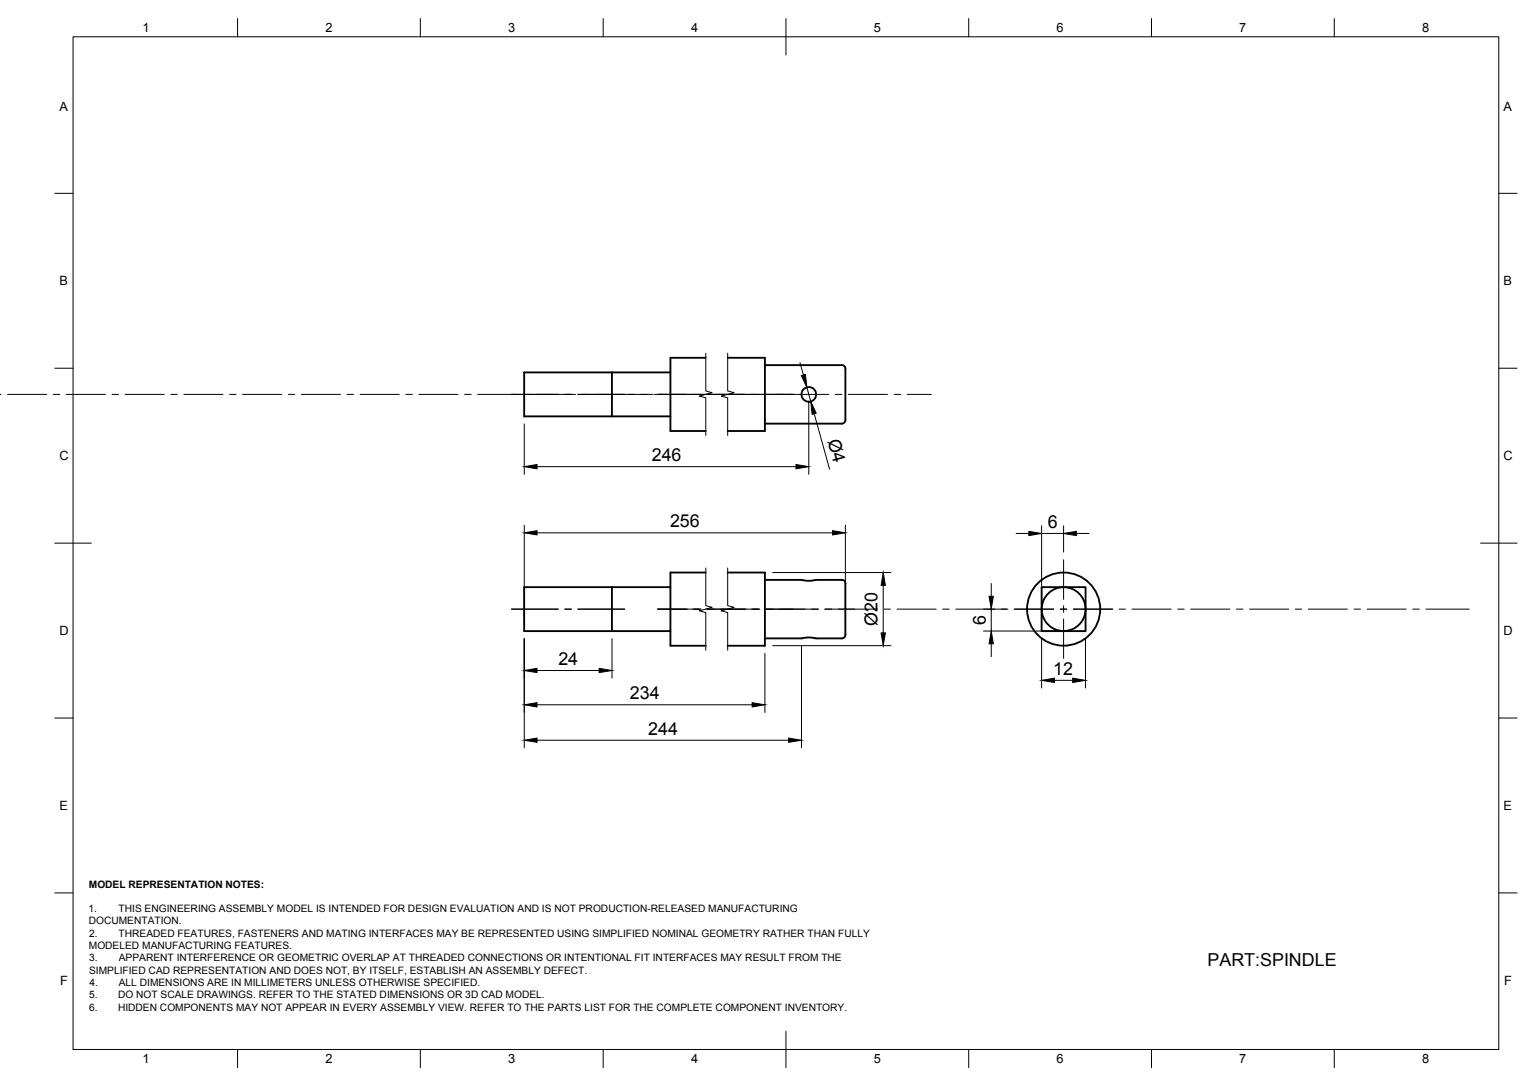
ISO-10303-21;
HEADER;
/* Generated by software containing ST-Developer
 * from STEP Tools, Inc. (www.steptools.com) 
 */

FILE_DESCRIPTION(
/* description */ (''),
/* implementation_level */ '2;1');

FILE_NAME(
/* name */ 'SPINDLE.step',
/* time_stamp */ '2026-10-04T02:10:06-07:00',
/* author */ (''),
/* organization */ (''),
/* preprocessor_version */ 'ST-DEVELOPER v20.2',
/* originating_system */ 'Autodesk Translation Framework v15.15.0.0',
/* authorisation */ '');

FILE_SCHEMA (('AUTOMOTIVE_DESIGN { 1 0 10303 214 3 1 1 }'));
ENDSEC;

DATA;
#10=MECHANICAL_DESIGN_GEOMETRIC_PRESENTATION_REPRESENTATION('',(#143),#9668);
#121=SHAPE_REPRESENTATION_RELATIONSHIP('SRR','None',#9714,#132);
#132=ADVANCED_BREP_SHAPE_REPRESENTATION('',(#154),#9659);
#143=STYLED_ITEM('',(#9775),#154);
#154=MANIFOLD_SOLID_BREP('Body1',#3883);
#233=FACE_BOUND('',#1154,.T.);
#234=FACE_BOUND('',#1157,.T.);
#235=FACE_BOUND('',#1159,.T.);
#236=FACE_BOUND('',#1160,.T.);
#299=PLANE('',#4195);
#300=PLANE('',#4197);
#301=PLANE('',#4199);
#302=PLANE('',#4201);
#303=PLANE('',#4203);
#304=PLANE('',#4207);
#305=PLANE('',#4214);
#306=PLANE('',#4215);
#307=PLANE('',#4216);
#308=PLANE('',#4217);
#309=PLANE('',#4218);
#310=PLANE('',#4222);
#446=LINE('',#6435,#637);
#447=LINE('',#6436,#638);
#448=LINE('',#6441,#639);
#449=LINE('',#6442,#640);
#450=LINE('',#6447,#641);
#451=LINE('',#6448,#642);
#452=LINE('',#6457,#643);
#453=LINE('',#6459,#644);
#454=LINE('',#6461,#645);
#455=LINE('',#6462,#646);
#456=LINE('',#6466,#647);
#457=LINE('',#6473,#648);
#458=LINE('',#6551,#649);
#459=LINE('',#6555,#650);
#460=LINE('',#6557,#651);
#461=LINE('',#6558,#652);
#462=LINE('',#6560,#653);
#463=LINE('',#6562,#654);
#464=LINE('',#6564,#655);
#465=LINE('',#6569,#656);
#637=VECTOR('',#4910,6.);
#638=VECTOR('',#4911,6.);
#639=VECTOR('',#4916,6.);
#640=VECTOR('',#4917,6.);
#641=VECTOR('',#4922,6.);
#642=VECTOR('',#4923,6.);
#643=VECTOR('',#4932,12.);
#644=VECTOR('',#4933,12.);
#645=VECTOR('',#4934,12.);
#646=VECTOR('',#4935,12.);
#647=VECTOR('',#4940,9.99999999999998);
#648=VECTOR('',#4949,8.);
#649=VECTOR('',#4952,2.);
#650=VECTOR('',#4959,16.);
#651=VECTOR('',#4960,6.);
#652=VECTOR('',#4961,16.);
#653=VECTOR('',#4964,16.);
#654=VECTOR('',#4967,16.);
#655=VECTOR('',#4970,6.);
#656=VECTOR('',#4977,6.);
#786=CYLINDRICAL_SURFACE('',#4205,9.99999999999998);
#787=CYLINDRICAL_SURFACE('',#4209,8.);
#788=CYLINDRICAL_SURFACE('',#4211,2.);
#789=CYLINDRICAL_SURFACE('',#4220,6.);
#888=FACE_OUTER_BOUND('',#1149,.T.);
#889=FACE_OUTER_BOUND('',#1150,.T.);
#890=FACE_OUTER_BOUND('',#1151,.T.);
#891=FACE_OUTER_BOUND('',#1152,.T.);
#892=FACE_OUTER_BOUND('',#1153,.T.);
#893=FACE_OUTER_BOUND('',#1155,.T.);
#894=FACE_OUTER_BOUND('',#1156,.T.);
#895=FACE_OUTER_BOUND('',#1158,.T.);
#896=FACE_OUTER_BOUND('',#1161,.T.);
#897=FACE_OUTER_BOUND('',#1162,.T.);
#898=FACE_OUTER_BOUND('',#1163,.T.);
#899=FACE_OUTER_BOUND('',#1164,.T.);
#900=FACE_OUTER_BOUND('',#1165,.T.);
#901=FACE_OUTER_BOUND('',#1166,.T.);
#902=FACE_OUTER_BOUND('',#1167,.T.);
#903=FACE_OUTER_BOUND('',#1168,.T.);
#904=FACE_OUTER_BOUND('',#1169,.T.);
#1149=EDGE_LOOP('',(#2933,#2934,#2935));
#1150=EDGE_LOOP('',(#2936,#2937,#2938));
#1151=EDGE_LOOP('',(#2939,#2940,#2941));
#1152=EDGE_LOOP('',(#2942));
#1153=EDGE_LOOP('',(#2943));
#1154=EDGE_LOOP('',(#2944,#2945,#2946,#2947));
#1155=EDGE_LOOP('',(#2948,#2949,#2950,#2951));
#1156=EDGE_LOOP('',(#2952));
#1157=EDGE_LOOP('',(#2953));
#1158=EDGE_LOOP('',(#2954,#2955,#2956,#2957));
#1159=EDGE_LOOP('',(#2958,#2959));
#1160=EDGE_LOOP('',(#2960,#2961));
#1161=EDGE_LOOP('',(#2962,#2963,#2964,#2965,#2966,#2967));
#1162=EDGE_LOOP('',(#2968,#2969,#2970,#2971));
#1163=EDGE_LOOP('',(#2972,#2973,#2974,#2975,#2976));
#1164=EDGE_LOOP('',(#2977,#2978,#2979,#2980,#2981));
#1165=EDGE_LOOP('',(#2982,#2983,#2984,#2985,#2986));
#1166=EDGE_LOOP('',(#2987,#2988,#2989,#2990,#2991));
#1167=EDGE_LOOP('',(#2992,#2993,#2994));
#1168=EDGE_LOOP('',(#2995,#2996,#2997,#2998,#2999,#3000,#3001));
#1169=EDGE_LOOP('',(#3002));
#1343=B_SPLINE_CURVE_WITH_KNOTS('',3,(#6476,#6477,#6478,#6479,#6480,#6481,
#6482,#6483,#6484,#6485,#6486,#6487,#6488,#6489,#6490,#6491,#6492,#6493),
 .UNSPECIFIED.,.F.,.F.,(4,2,2,2,2,2,2,2,4),(0.605474840211907,0.681164486618941,
0.756854133025976,0.832533196671918,0.90821226031786,0.983891323963802,
1.05957038760974,1.13526003401678,1.21094968042381),.UNSPECIFIED.);
#1344=B_SPLINE_CURVE_WITH_KNOTS('',3,(#6494,#6495,#6496,#6497,#6498,#6499,
#6500,#6501,#6502,#6503,#6504,#6505,#6506,#6507,#6508,#6509,#6510,#6511),
 .UNSPECIFIED.,.F.,.F.,(4,2,2,2,2,2,2,2,4),(1.21094968042381,1.28663932683085,
1.36232897323788,1.43800803688382,1.51368710052977,1.58936616417571,1.66504522782165,
1.74073487422869,1.81642452063572),.UNSPECIFIED.);
#1345=B_SPLINE_CURVE_WITH_KNOTS('',3,(#6514,#6515,#6516,#6517,#6518,#6519,
#6520,#6521,#6522,#6523,#6524,#6525,#6526,#6527,#6528,#6529,#6530,#6531),
 .UNSPECIFIED.,.F.,.F.,(4,2,2,2,2,2,2,2,4),(0.605474840211907,0.681164486618941,
0.756854133025976,0.832533196671918,0.90821226031786,0.983891323963802,
1.05957038760974,1.13526003401678,1.21094968042381),.UNSPECIFIED.);
#1346=B_SPLINE_CURVE_WITH_KNOTS('',3,(#6532,#6533,#6534,#6535,#6536,#6537,
#6538,#6539,#6540,#6541,#6542,#6543,#6544,#6545,#6546,#6547,#6548,#6549),
 .UNSPECIFIED.,.F.,.F.,(4,2,2,2,2,2,2,2,4),(1.21094968042381,1.28663932683085,
1.36232897323788,1.43800803688382,1.51368710052977,1.58936616417571,1.66504522782165,
1.74073487422869,1.81642452063572),.UNSPECIFIED.);
#1526=CIRCLE('',#4196,6.);
#1527=CIRCLE('',#4198,6.);
#1528=CIRCLE('',#4200,6.);
#1529=CIRCLE('',#4202,7.);
#1530=CIRCLE('',#4204,9.99999999999995);
#1531=CIRCLE('',#4206,10.);
#1532=CIRCLE('',#4208,7.99999999999999);
#1533=CIRCLE('',#4210,8.);
#1534=CIRCLE('',#4213,1.);
#1535=CIRCLE('',#4219,6.);
#1536=CIRCLE('',#4221,6.);
#1769=VERTEX_POINT('',#6431);
#1770=VERTEX_POINT('',#6432);
#1771=VERTEX_POINT('',#6434);
#1772=VERTEX_POINT('',#6438);
#1773=VERTEX_POINT('',#6440);
#1774=VERTEX_POINT('',#6444);
#1775=VERTEX_POINT('',#6446);
#1776=VERTEX_POINT('',#6450);
#1777=VERTEX_POINT('',#6453);
#1778=VERTEX_POINT('',#6455);
#1779=VERTEX_POINT('',#6456);
#1780=VERTEX_POINT('',#6458);
#1781=VERTEX_POINT('',#6460);
#1782=VERTEX_POINT('',#6464);
#1783=VERTEX_POINT('',#6468);
#1784=VERTEX_POINT('',#6471);
#1785=VERTEX_POINT('',#6474);
#1786=VERTEX_POINT('',#6475);
#1787=VERTEX_POINT('',#6512);
#1788=VERTEX_POINT('',#6513);
#1789=VERTEX_POINT('',#6556);
#1790=VERTEX_POINT('',#6568);
#2190=EDGE_CURVE('',#1769,#1770,#1526,.T.);
#2191=EDGE_CURVE('',#1769,#1771,#446,.T.);
#2192=EDGE_CURVE('',#1771,#1770,#447,.T.);
#2193=EDGE_CURVE('',#1770,#1772,#1527,.T.);
#2194=EDGE_CURVE('',#1770,#1773,#448,.T.);
#2195=EDGE_CURVE('',#1773,#1772,#449,.T.);
#2196=EDGE_CURVE('',#1772,#1774,#1528,.T.);
#2197=EDGE_CURVE('',#1772,#1775,#450,.T.);
#2198=EDGE_CURVE('',#1775,#1774,#451,.T.);
#2199=EDGE_CURVE('',#1776,#1776,#1529,.T.);
#2200=EDGE_CURVE('',#1777,#1777,#1530,.T.);
#2201=EDGE_CURVE('',#1778,#1779,#452,.T.);
#2202=EDGE_CURVE('',#1780,#1778,#453,.T.);
#2203=EDGE_CURVE('',#1781,#1780,#454,.T.);
#2204=EDGE_CURVE('',#1779,#1781,#455,.T.);
#2205=EDGE_CURVE('',#1782,#1782,#1531,.T.);
#2206=EDGE_CURVE('',#1782,#1777,#456,.T.);
#2207=EDGE_CURVE('',#1783,#1783,#1532,.T.);
#2208=EDGE_CURVE('',#1784,#1784,#1533,.F.);
#2209=EDGE_CURVE('',#1784,#1783,#457,.T.);
#2210=EDGE_CURVE('',#1785,#1786,#1343,.T.);
#2211=EDGE_CURVE('',#1786,#1785,#1344,.T.);
#2212=EDGE_CURVE('',#1787,#1788,#1345,.T.);
#2213=EDGE_CURVE('',#1788,#1787,#1346,.T.);
#2214=EDGE_CURVE('',#1786,#1788,#458,.T.);
#2215=EDGE_CURVE('',#1776,#1784,#1534,.T.);
#2216=EDGE_CURVE('',#1771,#1779,#459,.T.);
#2217=EDGE_CURVE('',#1789,#1769,#460,.T.);
#2218=EDGE_CURVE('',#1789,#1778,#461,.T.);
#2219=EDGE_CURVE('',#1773,#1781,#462,.T.);
#2220=EDGE_CURVE('',#1775,#1780,#463,.T.);
#2221=EDGE_CURVE('',#1774,#1789,#464,.T.);
#2222=EDGE_CURVE('',#1774,#1769,#1535,.T.);
#2223=EDGE_CURVE('',#1769,#1790,#465,.T.);
#2224=EDGE_CURVE('',#1790,#1790,#1536,.T.);
#2933=ORIENTED_EDGE('',*,*,#2190,.F.);
#2934=ORIENTED_EDGE('',*,*,#2191,.T.);
#2935=ORIENTED_EDGE('',*,*,#2192,.T.);
#2936=ORIENTED_EDGE('',*,*,#2193,.F.);
#2937=ORIENTED_EDGE('',*,*,#2194,.T.);
#2938=ORIENTED_EDGE('',*,*,#2195,.T.);
#2939=ORIENTED_EDGE('',*,*,#2196,.F.);
#2940=ORIENTED_EDGE('',*,*,#2197,.T.);
#2941=ORIENTED_EDGE('',*,*,#2198,.T.);
#2942=ORIENTED_EDGE('',*,*,#2199,.T.);
#2943=ORIENTED_EDGE('',*,*,#2200,.F.);
#2944=ORIENTED_EDGE('',*,*,#2201,.F.);
#2945=ORIENTED_EDGE('',*,*,#2202,.F.);
#2946=ORIENTED_EDGE('',*,*,#2203,.F.);
#2947=ORIENTED_EDGE('',*,*,#2204,.F.);
#2948=ORIENTED_EDGE('',*,*,#2205,.F.);
#2949=ORIENTED_EDGE('',*,*,#2206,.T.);
#2950=ORIENTED_EDGE('',*,*,#2200,.T.);
#2951=ORIENTED_EDGE('',*,*,#2206,.F.);
#2952=ORIENTED_EDGE('',*,*,#2205,.T.);
#2953=ORIENTED_EDGE('',*,*,#2207,.F.);
#2954=ORIENTED_EDGE('',*,*,#2208,.T.);
#2955=ORIENTED_EDGE('',*,*,#2209,.T.);
#2956=ORIENTED_EDGE('',*,*,#2207,.T.);
#2957=ORIENTED_EDGE('',*,*,#2209,.F.);
#2958=ORIENTED_EDGE('',*,*,#2210,.F.);
#2959=ORIENTED_EDGE('',*,*,#2211,.F.);
#2960=ORIENTED_EDGE('',*,*,#2212,.F.);
#2961=ORIENTED_EDGE('',*,*,#2213,.F.);
#2962=ORIENTED_EDGE('',*,*,#2210,.T.);
#2963=ORIENTED_EDGE('',*,*,#2214,.T.);
#2964=ORIENTED_EDGE('',*,*,#2213,.T.);
#2965=ORIENTED_EDGE('',*,*,#2212,.T.);
#2966=ORIENTED_EDGE('',*,*,#2214,.F.);
#2967=ORIENTED_EDGE('',*,*,#2211,.T.);
#2968=ORIENTED_EDGE('',*,*,#2199,.F.);
#2969=ORIENTED_EDGE('',*,*,#2215,.T.);
#2970=ORIENTED_EDGE('',*,*,#2208,.F.);
#2971=ORIENTED_EDGE('',*,*,#2215,.F.);
#2972=ORIENTED_EDGE('',*,*,#2201,.T.);
#2973=ORIENTED_EDGE('',*,*,#2216,.F.);
#2974=ORIENTED_EDGE('',*,*,#2191,.F.);
#2975=ORIENTED_EDGE('',*,*,#2217,.F.);
#2976=ORIENTED_EDGE('',*,*,#2218,.T.);
#2977=ORIENTED_EDGE('',*,*,#2204,.T.);
#2978=ORIENTED_EDGE('',*,*,#2219,.F.);
#2979=ORIENTED_EDGE('',*,*,#2194,.F.);
#2980=ORIENTED_EDGE('',*,*,#2192,.F.);
#2981=ORIENTED_EDGE('',*,*,#2216,.T.);
#2982=ORIENTED_EDGE('',*,*,#2203,.T.);
#2983=ORIENTED_EDGE('',*,*,#2220,.F.);
#2984=ORIENTED_EDGE('',*,*,#2197,.F.);
#2985=ORIENTED_EDGE('',*,*,#2195,.F.);
#2986=ORIENTED_EDGE('',*,*,#2219,.T.);
#2987=ORIENTED_EDGE('',*,*,#2202,.T.);
#2988=ORIENTED_EDGE('',*,*,#2218,.F.);
#2989=ORIENTED_EDGE('',*,*,#2221,.F.);
#2990=ORIENTED_EDGE('',*,*,#2198,.F.);
#2991=ORIENTED_EDGE('',*,*,#2220,.T.);
#2992=ORIENTED_EDGE('',*,*,#2222,.F.);
#2993=ORIENTED_EDGE('',*,*,#2221,.T.);
#2994=ORIENTED_EDGE('',*,*,#2217,.T.);
#2995=ORIENTED_EDGE('',*,*,#2190,.T.);
#2996=ORIENTED_EDGE('',*,*,#2193,.T.);
#2997=ORIENTED_EDGE('',*,*,#2196,.T.);
#2998=ORIENTED_EDGE('',*,*,#2222,.T.);
#2999=ORIENTED_EDGE('',*,*,#2223,.T.);
#3000=ORIENTED_EDGE('',*,*,#2224,.F.);
#3001=ORIENTED_EDGE('',*,*,#2223,.F.);
#3002=ORIENTED_EDGE('',*,*,#2224,.T.);
#3642=TOROIDAL_SURFACE('',#4212,7.,1.);
#3736=ADVANCED_FACE('',(#888),#299,.T.);
#3737=ADVANCED_FACE('',(#889),#300,.T.);
#3738=ADVANCED_FACE('',(#890),#301,.T.);
#3739=ADVANCED_FACE('',(#891),#302,.T.);
#3740=ADVANCED_FACE('',(#892,#233),#303,.T.);
#3741=ADVANCED_FACE('',(#893),#786,.T.);
#3742=ADVANCED_FACE('',(#894,#234),#304,.T.);
#3743=ADVANCED_FACE('',(#895,#235,#236),#787,.T.);
#3744=ADVANCED_FACE('',(#896),#788,.F.);
#3745=ADVANCED_FACE('',(#897),#3642,.T.);
#3746=ADVANCED_FACE('',(#898),#305,.F.);
#3747=ADVANCED_FACE('',(#899),#306,.F.);
#3748=ADVANCED_FACE('',(#900),#307,.F.);
#3749=ADVANCED_FACE('',(#901),#308,.F.);
#3750=ADVANCED_FACE('',(#902),#309,.T.);
#3751=ADVANCED_FACE('',(#903),#789,.T.);
#3752=ADVANCED_FACE('',(#904),#310,.T.);
#3883=CLOSED_SHELL('',(#3736,#3737,#3738,#3739,#3740,#3741,#3742,#3743,
#3744,#3745,#3746,#3747,#3748,#3749,#3750,#3751,#3752));
#4194=AXIS2_PLACEMENT_3D('',#6429,#4904,#4905);
#4195=AXIS2_PLACEMENT_3D('',#6430,#4906,#4907);
#4196=AXIS2_PLACEMENT_3D('',#6433,#4908,#4909);
#4197=AXIS2_PLACEMENT_3D('',#6437,#4912,#4913);
#4198=AXIS2_PLACEMENT_3D('',#6439,#4914,#4915);
#4199=AXIS2_PLACEMENT_3D('',#6443,#4918,#4919);
#4200=AXIS2_PLACEMENT_3D('',#6445,#4920,#4921);
#4201=AXIS2_PLACEMENT_3D('',#6449,#4924,#4925);
#4202=AXIS2_PLACEMENT_3D('',#6451,#4926,#4927);
#4203=AXIS2_PLACEMENT_3D('',#6452,#4928,#4929);
#4204=AXIS2_PLACEMENT_3D('',#6454,#4930,#4931);
#4205=AXIS2_PLACEMENT_3D('',#6463,#4936,#4937);
#4206=AXIS2_PLACEMENT_3D('',#6465,#4938,#4939);
#4207=AXIS2_PLACEMENT_3D('',#6467,#4941,#4942);
#4208=AXIS2_PLACEMENT_3D('',#6469,#4943,#4944);
#4209=AXIS2_PLACEMENT_3D('',#6470,#4945,#4946);
#4210=AXIS2_PLACEMENT_3D('',#6472,#4947,#4948);
#4211=AXIS2_PLACEMENT_3D('',#6550,#4950,#4951);
#4212=AXIS2_PLACEMENT_3D('',#6552,#4953,#4954);
#4213=AXIS2_PLACEMENT_3D('',#6553,#4955,#4956);
#4214=AXIS2_PLACEMENT_3D('',#6554,#4957,#4958);
#4215=AXIS2_PLACEMENT_3D('',#6559,#4962,#4963);
#4216=AXIS2_PLACEMENT_3D('',#6561,#4965,#4966);
#4217=AXIS2_PLACEMENT_3D('',#6563,#4968,#4969);
#4218=AXIS2_PLACEMENT_3D('',#6565,#4971,#4972);
#4219=AXIS2_PLACEMENT_3D('',#6566,#4973,#4974);
#4220=AXIS2_PLACEMENT_3D('',#6567,#4975,#4976);
#4221=AXIS2_PLACEMENT_3D('',#6570,#4978,#4979);
#4222=AXIS2_PLACEMENT_3D('',#6571,#4980,#4981);
#4904=DIRECTION('axis',(0.,0.,1.));
#4905=DIRECTION('refdir',(1.,0.,0.));
#4906=DIRECTION('center_axis',(1.,0.,0.));
#4907=DIRECTION('ref_axis',(0.,0.,-1.));
#4908=DIRECTION('center_axis',(1.,0.,0.));
#4909=DIRECTION('ref_axis',(0.,0.,-1.));
#4910=DIRECTION('',(0.,1.,1.85037170770859E-16));
#4911=DIRECTION('',(0.,0.,1.));
#4912=DIRECTION('center_axis',(1.,0.,0.));
#4913=DIRECTION('ref_axis',(0.,0.,-1.));
#4914=DIRECTION('center_axis',(1.,0.,0.));
#4915=DIRECTION('ref_axis',(0.,0.,-1.));
#4916=DIRECTION('',(0.,0.,1.));
#4917=DIRECTION('',(0.,-1.,-1.85037170770859E-16));
#4918=DIRECTION('center_axis',(1.,0.,0.));
#4919=DIRECTION('ref_axis',(0.,0.,-1.));
#4920=DIRECTION('center_axis',(1.,0.,0.));
#4921=DIRECTION('ref_axis',(0.,0.,-1.));
#4922=DIRECTION('',(0.,-1.,-1.8503717077086E-16));
#4923=DIRECTION('',(0.,0.,-1.));
#4924=DIRECTION('center_axis',(-1.,0.,0.));
#4925=DIRECTION('ref_axis',(0.,0.,1.));
#4926=DIRECTION('center_axis',(-1.,0.,0.));
#4927=DIRECTION('ref_axis',(0.,0.,1.));
#4928=DIRECTION('center_axis',(1.,0.,0.));
#4929=DIRECTION('ref_axis',(0.,0.,-1.));
#4930=DIRECTION('center_axis',(-1.,0.,0.));
#4931=DIRECTION('ref_axis',(0.,0.,1.));
#4932=DIRECTION('',(0.,1.,9.25185853854297E-17));
#4933=DIRECTION('',(0.,9.25185853854297E-17,-1.));
#4934=DIRECTION('',(0.,-1.,-1.85037170770859E-16));
#4935=DIRECTION('',(0.,0.,1.));
#4936=DIRECTION('center_axis',(-1.,0.,0.));
#4937=DIRECTION('ref_axis',(0.,0.,1.));
#4938=DIRECTION('center_axis',(-1.,0.,0.));
#4939=DIRECTION('ref_axis',(0.,0.,1.));
#4940=DIRECTION('',(1.,0.,0.));
#4941=DIRECTION('center_axis',(-1.,0.,0.));
#4942=DIRECTION('ref_axis',(0.,0.,1.));
#4943=DIRECTION('center_axis',(-1.,0.,0.));
#4944=DIRECTION('ref_axis',(0.,0.,1.));
#4945=DIRECTION('center_axis',(-1.,0.,0.));
#4946=DIRECTION('ref_axis',(0.,0.,1.));
#4947=DIRECTION('center_axis',(-1.,0.,0.));
#4948=DIRECTION('ref_axis',(0.,0.,1.));
#4949=DIRECTION('',(1.,0.,0.));
#4950=DIRECTION('center_axis',(0.,1.,0.));
#4951=DIRECTION('ref_axis',(0.,0.,1.));
#4952=DIRECTION('',(0.,1.,0.));
#4953=DIRECTION('center_axis',(-1.,0.,0.));
#4954=DIRECTION('ref_axis',(0.,0.,1.));
#4955=DIRECTION('center_axis',(0.,-1.,1.22464679914735E-16));
#4956=DIRECTION('ref_axis',(0.,-1.22464679914735E-16,-1.));
#4957=DIRECTION('center_axis',(0.,-1.44560289664734E-16,1.));
#4958=DIRECTION('ref_axis',(1.,0.,0.));
#4959=DIRECTION('',(-1.,0.,0.));
#4960=DIRECTION('',(0.,1.,0.));
#4961=DIRECTION('',(-1.,0.,0.));
#4962=DIRECTION('center_axis',(0.,-1.,0.));
#4963=DIRECTION('ref_axis',(0.,0.,-1.));
#4964=DIRECTION('',(-1.,0.,0.));
#4965=DIRECTION('center_axis',(0.,1.44560289664734E-16,-1.));
#4966=DIRECTION('ref_axis',(-1.,0.,0.));
#4967=DIRECTION('',(-1.,0.,0.));
#4968=DIRECTION('center_axis',(0.,1.,1.44560289664734E-16));
#4969=DIRECTION('ref_axis',(0.,-1.44560289664734E-16,1.));
#4970=DIRECTION('',(0.,1.85037170770859E-16,-1.));
#4971=DIRECTION('center_axis',(1.,0.,0.));
#4972=DIRECTION('ref_axis',(0.,0.,-1.));
#4973=DIRECTION('center_axis',(1.,0.,0.));
#4974=DIRECTION('ref_axis',(0.,0.,-1.));
#4975=DIRECTION('center_axis',(-1.,0.,0.));
#4976=DIRECTION('ref_axis',(0.,0.,1.));
#4977=DIRECTION('',(1.,0.,0.));
#4978=DIRECTION('center_axis',(1.,0.,0.));
#4979=DIRECTION('ref_axis',(0.,0.,-1.));
#4980=DIRECTION('center_axis',(1.,0.,0.));
#4981=DIRECTION('ref_axis',(0.,0.,-1.));
#6429=CARTESIAN_POINT('',(0.,0.,0.));
#6430=CARTESIAN_POINT('Origin',(232.,0.,0.));
#6431=CARTESIAN_POINT('',(232.,8.67361737988404E-16,-6.));
#6432=CARTESIAN_POINT('',(232.,6.,0.));
#6433=CARTESIAN_POINT('Origin',(232.,0.,0.));
#6434=CARTESIAN_POINT('',(232.,6.,-6.));
#6435=CARTESIAN_POINT('',(232.,8.67361737988404E-16,-6.));
#6436=CARTESIAN_POINT('',(232.,6.,-6.));
#6437=CARTESIAN_POINT('Origin',(232.,0.,0.));
#6438=CARTESIAN_POINT('',(232.,-8.67361737988403E-16,6.));
#6439=CARTESIAN_POINT('Origin',(232.,0.,0.));
#6440=CARTESIAN_POINT('',(232.,6.,6.));
#6441=CARTESIAN_POINT('',(232.,6.,0.));
#6442=CARTESIAN_POINT('',(232.,6.,6.));
#6443=CARTESIAN_POINT('Origin',(232.,0.,0.));
#6444=CARTESIAN_POINT('',(232.,-6.,-8.67361737988403E-16));
#6445=CARTESIAN_POINT('Origin',(232.,0.,0.));
#6446=CARTESIAN_POINT('',(232.,-6.,6.));
#6447=CARTESIAN_POINT('',(232.,8.67361737988404E-16,6.));
#6448=CARTESIAN_POINT('',(232.,-6.,6.));
#6449=CARTESIAN_POINT('Origin',(0.,-8.,0.));
#6450=CARTESIAN_POINT('',(0.,-8.57252759403147E-16,-7.));
#6451=CARTESIAN_POINT('Origin',(0.,0.,0.));
#6452=CARTESIAN_POINT('Origin',(216.,0.,0.));
#6453=CARTESIAN_POINT('',(216.,-1.22464679914735E-15,-9.99999999999998));
#6454=CARTESIAN_POINT('Origin',(216.,0.,0.));
#6455=CARTESIAN_POINT('',(216.,-6.,-6.));
#6456=CARTESIAN_POINT('',(216.,6.,-6.));
#6457=CARTESIAN_POINT('',(216.,-6.,-6.));
#6458=CARTESIAN_POINT('',(216.,-6.,6.));
#6459=CARTESIAN_POINT('',(216.,-6.,6.));
#6460=CARTESIAN_POINT('',(216.,6.,6.));
#6461=CARTESIAN_POINT('',(216.,6.,6.));
#6462=CARTESIAN_POINT('',(216.,6.,-6.));
#6463=CARTESIAN_POINT('Origin',(0.,0.,0.));
#6464=CARTESIAN_POINT('',(22.,-1.22464679914735E-15,-9.99999999999998));
#6465=CARTESIAN_POINT('Origin',(22.,0.,0.));
#6466=CARTESIAN_POINT('',(0.,-1.22464679914735E-15,-9.99999999999998));
#6467=CARTESIAN_POINT('Origin',(22.,-10.,0.));
#6468=CARTESIAN_POINT('',(22.,-9.79717439317882E-16,-8.));
#6469=CARTESIAN_POINT('Origin',(22.,0.,0.));
#6470=CARTESIAN_POINT('Origin',(0.,0.,0.));
#6471=CARTESIAN_POINT('',(1.,-9.79717439317882E-16,-8.));
#6472=CARTESIAN_POINT('Origin',(1.,0.,0.));
#6473=CARTESIAN_POINT('',(0.,-9.79717439317882E-16,-8.));
#6474=CARTESIAN_POINT('',(10.,-7.74596669241483,2.));
#6475=CARTESIAN_POINT('',(10.,-7.74596669241483,-2.));
#6476=CARTESIAN_POINT('Ctrl Pts',(10.,-7.74596669241483,2.));
#6477=CARTESIAN_POINT('Ctrl Pts',(9.74770117864322,-7.74596669241483,2.));
#6478=CARTESIAN_POINT('Ctrl Pts',(9.479356583979,-7.75957726931369,1.94935810817991));
#6479=CARTESIAN_POINT('Ctrl Pts',(8.98693862993913,-7.8080895555786,1.74492797023227));
#6480=CARTESIAN_POINT('Ctrl Pts',(8.76276709090545,-7.84222121032682,1.59119421565164));
#6481=CARTESIAN_POINT('Ctrl Pts',(8.40883052939687,-7.90579009335489,1.23725765414306));
#6482=CARTESIAN_POINT('Ctrl Pts',(8.25507748138546,-7.93945007560673,1.01307580920409));
#6483=CARTESIAN_POINT('Ctrl Pts',(8.05063325793989,-7.98687320195912,0.520621311632992));
#6484=CARTESIAN_POINT('Ctrl Pts',(8.,-8.,0.252263545486474));
#6485=CARTESIAN_POINT('Ctrl Pts',(8.,-8.,-0.252263545486473));
#6486=CARTESIAN_POINT('Ctrl Pts',(8.05063325793989,-7.98687320195912,-0.52062131163299));
#6487=CARTESIAN_POINT('Ctrl Pts',(8.25507748138546,-7.93945007560673,-1.01307580920409));
#6488=CARTESIAN_POINT('Ctrl Pts',(8.40883052939687,-7.90579009335489,-1.23725765414306));
#6489=CARTESIAN_POINT('Ctrl Pts',(8.76276709090545,-7.84222121032682,-1.59119421565164));
#6490=CARTESIAN_POINT('Ctrl Pts',(8.98693862993913,-7.8080895555786,-1.74492797023227));
#6491=CARTESIAN_POINT('Ctrl Pts',(9.479356583979,-7.75957726931369,-1.94935810817991));
#6492=CARTESIAN_POINT('Ctrl Pts',(9.74770117864322,-7.74596669241483,-2.));
#6493=CARTESIAN_POINT('Ctrl Pts',(10.,-7.74596669241483,-2.));
#6494=CARTESIAN_POINT('Ctrl Pts',(10.,-7.74596669241483,-2.));
#6495=CARTESIAN_POINT('Ctrl Pts',(10.2522988213568,-7.74596669241483,-2.));
#6496=CARTESIAN_POINT('Ctrl Pts',(10.520643416021,-7.75957726931369,-1.94935810817991));
#6497=CARTESIAN_POINT('Ctrl Pts',(11.0130613700609,-7.8080895555786,-1.74492797023227));
#6498=CARTESIAN_POINT('Ctrl Pts',(11.2372329090946,-7.84222121032682,-1.59119421565164));
#6499=CARTESIAN_POINT('Ctrl Pts',(11.5911694706031,-7.90579009335489,-1.23725765414306));
#6500=CARTESIAN_POINT('Ctrl Pts',(11.7449225186145,-7.93945007560673,-1.01307580920409));
#6501=CARTESIAN_POINT('Ctrl Pts',(11.9493667420601,-7.98687320195912,-0.520621311632991));
#6502=CARTESIAN_POINT('Ctrl Pts',(12.,-8.,-0.252263545486473));
#6503=CARTESIAN_POINT('Ctrl Pts',(12.,-8.,0.252263545486474));
#6504=CARTESIAN_POINT('Ctrl Pts',(11.9493667420601,-7.98687320195912,0.520621311632992));
#6505=CARTESIAN_POINT('Ctrl Pts',(11.7449225186145,-7.93945007560673,1.01307580920409));
#6506=CARTESIAN_POINT('Ctrl Pts',(11.5911694706031,-7.90579009335489,1.23725765414306));
#6507=CARTESIAN_POINT('Ctrl Pts',(11.2372329090946,-7.84222121032682,1.59119421565164));
#6508=CARTESIAN_POINT('Ctrl Pts',(11.0130613700609,-7.8080895555786,1.74492797023227));
#6509=CARTESIAN_POINT('Ctrl Pts',(10.520643416021,-7.75957726931369,1.94935810817991));
#6510=CARTESIAN_POINT('Ctrl Pts',(10.2522988213568,-7.74596669241483,2.));
#6511=CARTESIAN_POINT('Ctrl Pts',(10.,-7.74596669241483,2.));
#6512=CARTESIAN_POINT('',(10.,7.74596669241483,2.));
#6513=CARTESIAN_POINT('',(10.,7.74596669241483,-2.));
#6514=CARTESIAN_POINT('Ctrl Pts',(10.,7.74596669241483,2.));
#6515=CARTESIAN_POINT('Ctrl Pts',(10.2522988213568,7.74596669241483,2.));
#6516=CARTESIAN_POINT('Ctrl Pts',(10.520643416021,7.75957726931369,1.94935810817991));
#6517=CARTESIAN_POINT('Ctrl Pts',(11.0130613700609,7.8080895555786,1.74492797023227));
#6518=CARTESIAN_POINT('Ctrl Pts',(11.2372329090946,7.84222121032682,1.59119421565164));
#6519=CARTESIAN_POINT('Ctrl Pts',(11.5911694706031,7.90579009335489,1.23725765414306));
#6520=CARTESIAN_POINT('Ctrl Pts',(11.7449225186145,7.93945007560673,1.01307580920409));
#6521=CARTESIAN_POINT('Ctrl Pts',(11.9493667420601,7.98687320195912,0.520621311632992));
#6522=CARTESIAN_POINT('Ctrl Pts',(12.,8.,0.252263545486474));
#6523=CARTESIAN_POINT('Ctrl Pts',(12.,8.,-0.252263545486473));
#6524=CARTESIAN_POINT('Ctrl Pts',(11.9493667420601,7.98687320195912,-0.520621311632991));
#6525=CARTESIAN_POINT('Ctrl Pts',(11.7449225186145,7.93945007560673,-1.01307580920409));
#6526=CARTESIAN_POINT('Ctrl Pts',(11.5911694706031,7.90579009335489,-1.23725765414306));
#6527=CARTESIAN_POINT('Ctrl Pts',(11.2372329090946,7.84222121032682,-1.59119421565164));
#6528=CARTESIAN_POINT('Ctrl Pts',(11.0130613700609,7.8080895555786,-1.74492797023227));
#6529=CARTESIAN_POINT('Ctrl Pts',(10.520643416021,7.75957726931369,-1.94935810817991));
#6530=CARTESIAN_POINT('Ctrl Pts',(10.2522988213568,7.74596669241483,-2.));
#6531=CARTESIAN_POINT('Ctrl Pts',(10.,7.74596669241483,-2.));
#6532=CARTESIAN_POINT('Ctrl Pts',(10.,7.74596669241483,-2.));
#6533=CARTESIAN_POINT('Ctrl Pts',(9.74770117864322,7.74596669241483,-2.));
#6534=CARTESIAN_POINT('Ctrl Pts',(9.479356583979,7.75957726931369,-1.94935810817991));
#6535=CARTESIAN_POINT('Ctrl Pts',(8.98693862993913,7.8080895555786,-1.74492797023227));
#6536=CARTESIAN_POINT('Ctrl Pts',(8.76276709090545,7.84222121032682,-1.59119421565164));
#6537=CARTESIAN_POINT('Ctrl Pts',(8.40883052939687,7.90579009335489,-1.23725765414306));
#6538=CARTESIAN_POINT('Ctrl Pts',(8.25507748138546,7.93945007560673,-1.01307580920409));
#6539=CARTESIAN_POINT('Ctrl Pts',(8.05063325793989,7.98687320195912,-0.52062131163299));
#6540=CARTESIAN_POINT('Ctrl Pts',(8.,8.,-0.252263545486473));
#6541=CARTESIAN_POINT('Ctrl Pts',(8.,8.,0.252263545486474));
#6542=CARTESIAN_POINT('Ctrl Pts',(8.05063325793989,7.98687320195912,0.520621311632991));
#6543=CARTESIAN_POINT('Ctrl Pts',(8.25507748138546,7.93945007560673,1.01307580920409));
#6544=CARTESIAN_POINT('Ctrl Pts',(8.40883052939687,7.90579009335489,1.23725765414306));
#6545=CARTESIAN_POINT('Ctrl Pts',(8.76276709090545,7.84222121032682,1.59119421565164));
#6546=CARTESIAN_POINT('Ctrl Pts',(8.98693862993913,7.8080895555786,1.74492797023227));
#6547=CARTESIAN_POINT('Ctrl Pts',(9.479356583979,7.75957726931369,1.94935810817991));
#6548=CARTESIAN_POINT('Ctrl Pts',(9.74770117864322,7.74596669241483,2.));
#6549=CARTESIAN_POINT('Ctrl Pts',(10.,7.74596669241483,2.));
#6550=CARTESIAN_POINT('Origin',(10.,-10.,0.));
#6551=CARTESIAN_POINT('',(10.,-10.,-2.));
#6552=CARTESIAN_POINT('Origin',(1.,0.,0.));
#6553=CARTESIAN_POINT('Origin',(1.,-8.57252759403147E-16,-7.));
#6554=CARTESIAN_POINT('Origin',(232.,6.,-6.));
#6555=CARTESIAN_POINT('',(232.,6.,-6.));
#6556=CARTESIAN_POINT('',(232.,-6.,-6.));
#6557=CARTESIAN_POINT('',(232.,-6.,-6.));
#6558=CARTESIAN_POINT('',(232.,-6.,-6.));
#6559=CARTESIAN_POINT('Origin',(232.,6.,6.));
#6560=CARTESIAN_POINT('',(232.,6.,6.));
#6561=CARTESIAN_POINT('Origin',(232.,6.,6.));
#6562=CARTESIAN_POINT('',(232.,-6.,6.));
#6563=CARTESIAN_POINT('Origin',(232.,-6.,6.));
#6564=CARTESIAN_POINT('',(232.,-6.,-8.67361737988404E-16));
#6565=CARTESIAN_POINT('Origin',(232.,0.,0.));
#6566=CARTESIAN_POINT('Origin',(232.,0.,0.));
#6567=CARTESIAN_POINT('Origin',(256.,0.,0.));
#6568=CARTESIAN_POINT('',(256.,0.,-6.));
#6569=CARTESIAN_POINT('',(256.,-7.34788079488412E-16,-6.));
#6570=CARTESIAN_POINT('Origin',(256.,0.,0.));
#6571=CARTESIAN_POINT('Origin',(256.,0.,0.));
#9646=UNCERTAINTY_MEASURE_WITH_UNIT(LENGTH_MEASURE(0.01),#9669,
'DISTANCE_ACCURACY_VALUE',
'Maximum model space distance between geometric entities at asserted c
onnectivities');
#9655=UNCERTAINTY_MEASURE_WITH_UNIT(LENGTH_MEASURE(0.01),#9669,
'DISTANCE_ACCURACY_VALUE',
'Maximum model space distance between geometric entities at asserted c
onnectivities');
#9659=(
GEOMETRIC_REPRESENTATION_CONTEXT(3)
GLOBAL_UNCERTAINTY_ASSIGNED_CONTEXT((#9646))
GLOBAL_UNIT_ASSIGNED_CONTEXT((#9669,#9671,#9672))
REPRESENTATION_CONTEXT('','3D')
);
#9668=(
GEOMETRIC_REPRESENTATION_CONTEXT(3)
GLOBAL_UNCERTAINTY_ASSIGNED_CONTEXT((#9655))
GLOBAL_UNIT_ASSIGNED_CONTEXT((#9669,#9671,#9672))
REPRESENTATION_CONTEXT('','3D')
);
#9669=(
LENGTH_UNIT()
NAMED_UNIT(*)
SI_UNIT(.MILLI.,.METRE.)
);
#9671=(
NAMED_UNIT(*)
PLANE_ANGLE_UNIT()
SI_UNIT($,.RADIAN.)
);
#9672=(
NAMED_UNIT(*)
SI_UNIT($,.STERADIAN.)
SOLID_ANGLE_UNIT()
);
#9676=SHAPE_DEFINITION_REPRESENTATION(#9688,#9714);
#9688=PRODUCT_DEFINITION_SHAPE('',$,#9727);
#9714=SHAPE_REPRESENTATION('',(#4194),#9659);
#9723=PRODUCT_DEFINITION_CONTEXT('part definition',#9761,'design');
#9727=PRODUCT_DEFINITION('2026-10-04-08-13-48-882','SPINDLE',#9739,#9723);
#9739=PRODUCT_DEFINITION_FORMATION('',$,#9766);
#9761=APPLICATION_CONTEXT(
'Core Data for Automotive Mechanical Design Process');
#9762=PRODUCT_CONTEXT('part definition',#9761,'mechanical');
#9766=PRODUCT('2026-10-04-08-13-48-882','SPINDLE','PART',(#9762));
#9775=PRESENTATION_STYLE_ASSIGNMENT((#9776));
#9776=SURFACE_STYLE_USAGE(.BOTH.,#9777);
#9777=SURFACE_SIDE_STYLE('',(#9778));
#9778=SURFACE_STYLE_FILL_AREA(#9779);
#9779=FILL_AREA_STYLE('Steel - Satin',(#9780));
#9780=FILL_AREA_STYLE_COLOUR('Steel - Satin',#9781);
#9781=COLOUR_RGB('Steel - Satin', 0.09019608, 0.27058824, 0.51372549);
ENDSEC;
END-ISO-10303-21;
